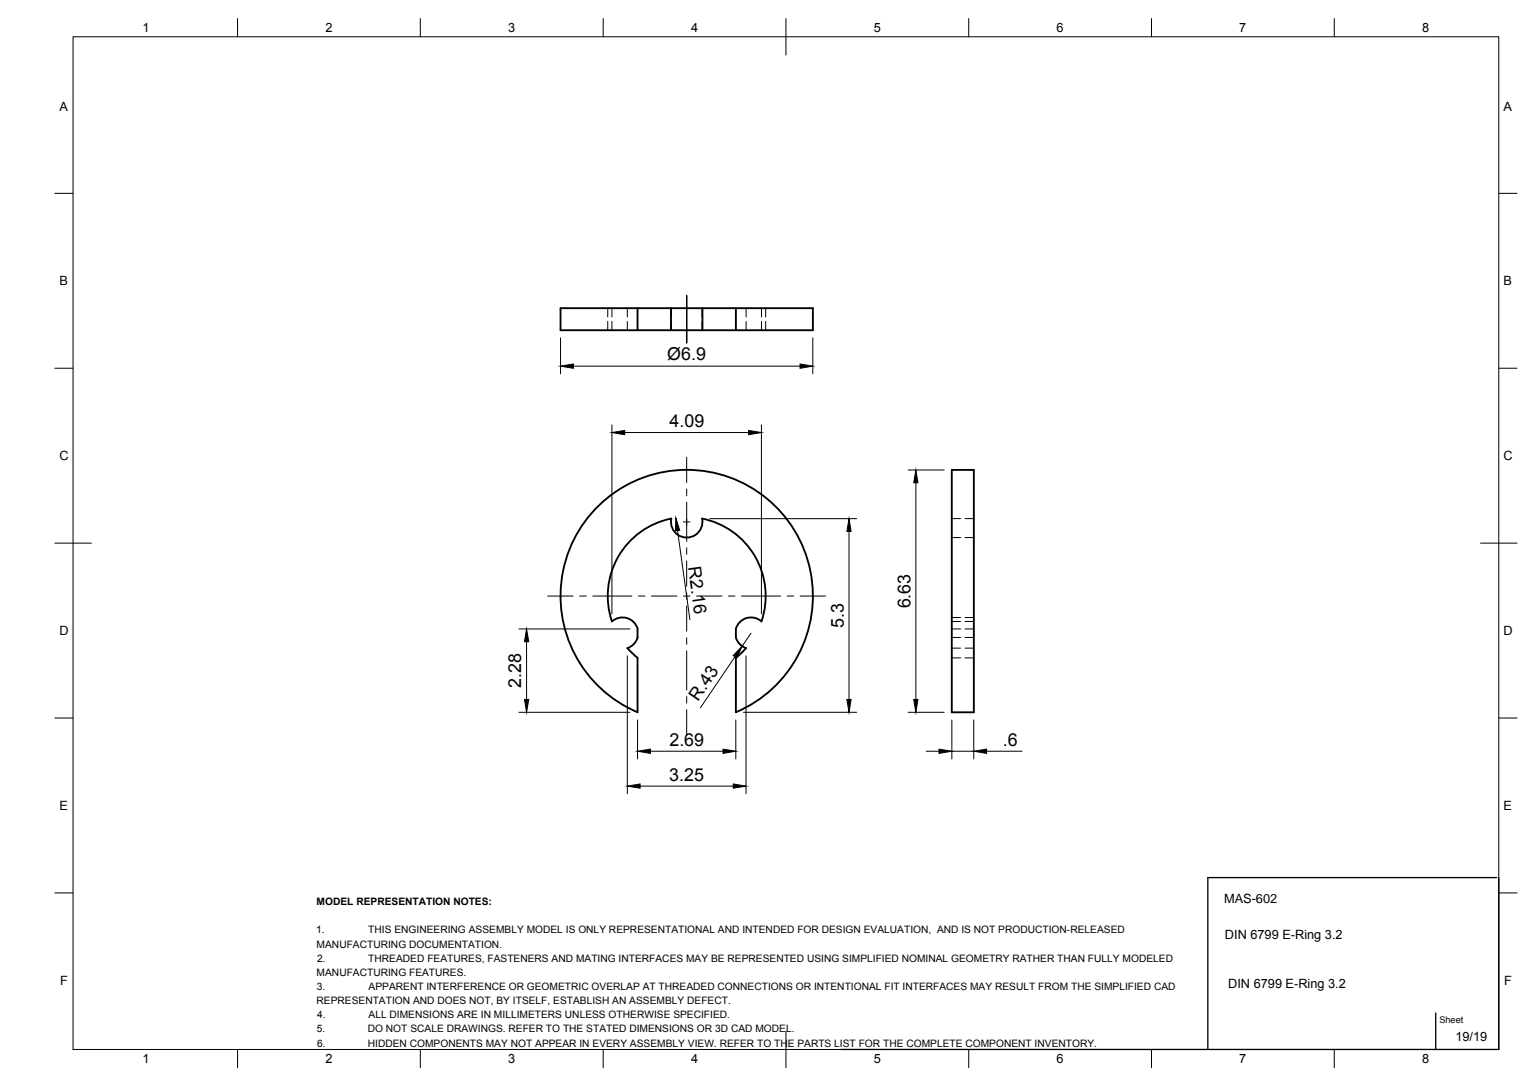
ISO-10303-21;
HEADER;
/* Generated by software containing ST-Developer
 * from STEP Tools, Inc. (www.steptools.com) 
 */

FILE_DESCRIPTION(
/* description */ (''),
/* implementation_level */ '2;1');

FILE_NAME(
/* name */ 'DIN 6799 E-Ring 3.2.step',
/* time_stamp */ '2026-10-15T14:42:47-07:00',
/* author */ (''),
/* organization */ (''),
/* preprocessor_version */ 'ST-DEVELOPER v20.2',
/* originating_system */ 'Autodesk Translation Framework v15.15.0.0',
/* authorisation */ '');

FILE_SCHEMA (('AUTOMOTIVE_DESIGN { 1 0 10303 214 3 1 1 }'));
ENDSEC;

DATA;
#10=MECHANICAL_DESIGN_GEOMETRIC_PRESENTATION_REPRESENTATION('',(#251),#85789);
#215=SHAPE_REPRESENTATION_RELATIONSHIP('SRR','None',#85880,#233);
#233=ADVANCED_BREP_SHAPE_REPRESENTATION('',(#269),#85788);
#251=STYLED_ITEM('',(#85978),#269);
#269=MANIFOLD_SOLID_BREP('Body1',#9898);
#1193=PLANE('',#10893);
#1194=PLANE('',#10894);
#1195=PLANE('',#10895);
#1196=PLANE('',#10896);
#1197=PLANE('',#10912);
#1198=PLANE('',#10928);
#1713=LINE('',#85637,#2249);
#1714=LINE('',#85639,#2250);
#1715=LINE('',#85641,#2251);
#1716=LINE('',#85642,#2252);
#1717=LINE('',#85646,#2253);
#1718=LINE('',#85648,#2254);
#1719=LINE('',#85650,#2255);
#1720=LINE('',#85651,#2256);
#1721=LINE('',#85655,#2257);
#1722=LINE('',#85657,#2258);
#1723=LINE('',#85659,#2259);
#1724=LINE('',#85660,#2260);
#1725=LINE('',#85664,#2261);
#1726=LINE('',#85666,#2262);
#1727=LINE('',#85668,#2263);
#1728=LINE('',#85669,#2264);
#1729=LINE('',#85674,#2265);
#1730=LINE('',#85680,#2266);
#1731=LINE('',#85686,#2267);
#1732=LINE('',#85692,#2268);
#1733=LINE('',#85710,#2269);
#1734=LINE('',#85714,#2270);
#2249=VECTOR('',#13065,1.);
#2250=VECTOR('',#13066,1.);
#2251=VECTOR('',#13067,1.);
#2252=VECTOR('',#13068,1.);
#2253=VECTOR('',#13071,1.);
#2254=VECTOR('',#13072,1.);
#2255=VECTOR('',#13073,1.);
#2256=VECTOR('',#13074,1.);
#2257=VECTOR('',#13077,1.);
#2258=VECTOR('',#13078,1.);
#2259=VECTOR('',#13079,1.);
#2260=VECTOR('',#13080,1.);
#2261=VECTOR('',#13083,1.);
#2262=VECTOR('',#13084,1.);
#2263=VECTOR('',#13085,1.);
#2264=VECTOR('',#13086,1.);
#2265=VECTOR('',#13091,1.);
#2266=VECTOR('',#13098,1.);
#2267=VECTOR('',#13105,1.);
#2268=VECTOR('',#13112,1.);
#2269=VECTOR('',#13141,1.);
#2270=VECTOR('',#13146,1.);
#2392=CYLINDRICAL_SURFACE('',#10897,0.04298125);
#2393=CYLINDRICAL_SURFACE('',#10900,0.04298125);
#2394=CYLINDRICAL_SURFACE('',#10903,0.04298125);
#2395=CYLINDRICAL_SURFACE('',#10906,0.04298125);
#2396=CYLINDRICAL_SURFACE('',#10909,0.2159625);
#2397=CYLINDRICAL_SURFACE('',#10918,0.2159625);
#2398=CYLINDRICAL_SURFACE('',#10920,0.2159625);
#2399=CYLINDRICAL_SURFACE('',#10922,0.04298125);
#2400=CYLINDRICAL_SURFACE('',#10924,0.2159625);
#2401=CYLINDRICAL_SURFACE('',#10926,0.345);
#2887=FACE_OUTER_BOUND('',#3477,.T.);
#2888=FACE_OUTER_BOUND('',#3478,.T.);
#2889=FACE_OUTER_BOUND('',#3479,.T.);
#2890=FACE_OUTER_BOUND('',#3480,.T.);
#2891=FACE_OUTER_BOUND('',#3481,.T.);
#2892=FACE_OUTER_BOUND('',#3482,.T.);
#2893=FACE_OUTER_BOUND('',#3483,.T.);
#2894=FACE_OUTER_BOUND('',#3484,.T.);
#2895=FACE_OUTER_BOUND('',#3485,.T.);
#2896=FACE_OUTER_BOUND('',#3486,.T.);
#2897=FACE_OUTER_BOUND('',#3487,.T.);
#2898=FACE_OUTER_BOUND('',#3488,.T.);
#2899=FACE_OUTER_BOUND('',#3489,.T.);
#2900=FACE_OUTER_BOUND('',#3490,.T.);
#2901=FACE_OUTER_BOUND('',#3491,.T.);
#2902=FACE_OUTER_BOUND('',#3492,.T.);
#3477=EDGE_LOOP('',(#9291,#9292,#9293,#9294));
#3478=EDGE_LOOP('',(#9295,#9296,#9297,#9298));
#3479=EDGE_LOOP('',(#9299,#9300,#9301,#9302));
#3480=EDGE_LOOP('',(#9303,#9304,#9305,#9306));
#3481=EDGE_LOOP('',(#9307,#9308,#9309,#9310));
#3482=EDGE_LOOP('',(#9311,#9312,#9313,#9314));
#3483=EDGE_LOOP('',(#9315,#9316,#9317,#9318));
#3484=EDGE_LOOP('',(#9319,#9320,#9321,#9322));
#3485=EDGE_LOOP('',(#9323,#9324,#9325,#9326));
#3486=EDGE_LOOP('',(#9327,#9328,#9329,#9330,#9331,#9332,#9333,#9334,#9335,
#9336,#9337,#9338,#9339,#9340));
#3487=EDGE_LOOP('',(#9341,#9342,#9343,#9344));
#3488=EDGE_LOOP('',(#9345,#9346,#9347,#9348));
#3489=EDGE_LOOP('',(#9349,#9350,#9351,#9352));
#3490=EDGE_LOOP('',(#9353,#9354,#9355,#9356));
#3491=EDGE_LOOP('',(#9357,#9358,#9359,#9360));
#3492=EDGE_LOOP('',(#9361,#9362,#9363,#9364,#9365,#9366,#9367,#9368,#9369,
#9370,#9371,#9372,#9373,#9374));
#3875=CIRCLE('',#10898,0.04298125);
#3876=CIRCLE('',#10899,0.04298125);
#3877=CIRCLE('',#10901,0.04298125);
#3878=CIRCLE('',#10902,0.04298125);
#3879=CIRCLE('',#10904,0.04298125);
#3880=CIRCLE('',#10905,0.04298125);
#3881=CIRCLE('',#10907,0.04298125);
#3882=CIRCLE('',#10908,0.04298125);
#3883=CIRCLE('',#10910,0.2159625);
#3884=CIRCLE('',#10911,0.2159625);
#3885=CIRCLE('',#10913,0.2159625);
#3886=CIRCLE('',#10914,0.04298125);
#3887=CIRCLE('',#10915,0.2159625);
#3888=CIRCLE('',#10916,0.345);
#3889=CIRCLE('',#10917,0.2159625);
#3890=CIRCLE('',#10919,0.2159625);
#3891=CIRCLE('',#10921,0.2159625);
#3892=CIRCLE('',#10923,0.04298125);
#3893=CIRCLE('',#10925,0.2159625);
#3894=CIRCLE('',#10927,0.345);
#4907=VERTEX_POINT('',#85635);
#4908=VERTEX_POINT('',#85636);
#4909=VERTEX_POINT('',#85638);
#4910=VERTEX_POINT('',#85640);
#4911=VERTEX_POINT('',#85644);
#4912=VERTEX_POINT('',#85645);
#4913=VERTEX_POINT('',#85647);
#4914=VERTEX_POINT('',#85649);
#4915=VERTEX_POINT('',#85653);
#4916=VERTEX_POINT('',#85654);
#4917=VERTEX_POINT('',#85656);
#4918=VERTEX_POINT('',#85658);
#4919=VERTEX_POINT('',#85662);
#4920=VERTEX_POINT('',#85663);
#4921=VERTEX_POINT('',#85665);
#4922=VERTEX_POINT('',#85667);
#4923=VERTEX_POINT('',#85671);
#4924=VERTEX_POINT('',#85673);
#4925=VERTEX_POINT('',#85677);
#4926=VERTEX_POINT('',#85679);
#4927=VERTEX_POINT('',#85683);
#4928=VERTEX_POINT('',#85685);
#4929=VERTEX_POINT('',#85689);
#4930=VERTEX_POINT('',#85691);
#4931=VERTEX_POINT('',#85698);
#4932=VERTEX_POINT('',#85700);
#4933=VERTEX_POINT('',#85708);
#4934=VERTEX_POINT('',#85712);
#6373=EDGE_CURVE('',#4907,#4908,#1713,.T.);
#6374=EDGE_CURVE('',#4909,#4907,#1714,.T.);
#6375=EDGE_CURVE('',#4910,#4909,#1715,.T.);
#6376=EDGE_CURVE('',#4908,#4910,#1716,.T.);
#6377=EDGE_CURVE('',#4911,#4912,#1717,.T.);
#6378=EDGE_CURVE('',#4913,#4911,#1718,.T.);
#6379=EDGE_CURVE('',#4914,#4913,#1719,.T.);
#6380=EDGE_CURVE('',#4912,#4914,#1720,.T.);
#6381=EDGE_CURVE('',#4915,#4916,#1721,.T.);
#6382=EDGE_CURVE('',#4917,#4915,#1722,.T.);
#6383=EDGE_CURVE('',#4918,#4917,#1723,.T.);
#6384=EDGE_CURVE('',#4916,#4918,#1724,.T.);
#6385=EDGE_CURVE('',#4919,#4920,#1725,.T.);
#6386=EDGE_CURVE('',#4921,#4919,#1726,.T.);
#6387=EDGE_CURVE('',#4922,#4921,#1727,.T.);
#6388=EDGE_CURVE('',#4920,#4922,#1728,.T.);
#6389=EDGE_CURVE('',#4923,#4913,#3875,.T.);
#6390=EDGE_CURVE('',#4924,#4923,#1729,.T.);
#6391=EDGE_CURVE('',#4924,#4914,#3876,.T.);
#6392=EDGE_CURVE('',#4912,#4925,#3877,.T.);
#6393=EDGE_CURVE('',#4925,#4926,#1730,.T.);
#6394=EDGE_CURVE('',#4911,#4926,#3878,.T.);
#6395=EDGE_CURVE('',#4927,#4921,#3879,.T.);
#6396=EDGE_CURVE('',#4928,#4927,#1731,.T.);
#6397=EDGE_CURVE('',#4928,#4922,#3880,.T.);
#6398=EDGE_CURVE('',#4920,#4929,#3881,.T.);
#6399=EDGE_CURVE('',#4929,#4930,#1732,.T.);
#6400=EDGE_CURVE('',#4919,#4930,#3882,.T.);
#6401=EDGE_CURVE('',#4916,#4928,#3883,.T.);
#6402=EDGE_CURVE('',#4915,#4927,#3884,.T.);
#6403=EDGE_CURVE('',#4931,#4924,#3885,.T.);
#6404=EDGE_CURVE('',#4932,#4931,#3886,.T.);
#6405=EDGE_CURVE('',#4929,#4932,#3887,.T.);
#6406=EDGE_CURVE('',#4909,#4918,#3888,.T.);
#6407=EDGE_CURVE('',#4925,#4907,#3889,.T.);
#6408=EDGE_CURVE('',#4926,#4908,#3890,.T.);
#6409=EDGE_CURVE('',#4933,#4923,#3891,.T.);
#6410=EDGE_CURVE('',#4931,#4933,#1733,.T.);
#6411=EDGE_CURVE('',#4934,#4933,#3892,.T.);
#6412=EDGE_CURVE('',#4932,#4934,#1734,.T.);
#6413=EDGE_CURVE('',#4930,#4934,#3893,.T.);
#6414=EDGE_CURVE('',#4910,#4917,#3894,.T.);
#9291=ORIENTED_EDGE('',*,*,#6373,.F.);
#9292=ORIENTED_EDGE('',*,*,#6374,.F.);
#9293=ORIENTED_EDGE('',*,*,#6375,.F.);
#9294=ORIENTED_EDGE('',*,*,#6376,.F.);
#9295=ORIENTED_EDGE('',*,*,#6377,.F.);
#9296=ORIENTED_EDGE('',*,*,#6378,.F.);
#9297=ORIENTED_EDGE('',*,*,#6379,.F.);
#9298=ORIENTED_EDGE('',*,*,#6380,.F.);
#9299=ORIENTED_EDGE('',*,*,#6381,.F.);
#9300=ORIENTED_EDGE('',*,*,#6382,.F.);
#9301=ORIENTED_EDGE('',*,*,#6383,.F.);
#9302=ORIENTED_EDGE('',*,*,#6384,.F.);
#9303=ORIENTED_EDGE('',*,*,#6385,.F.);
#9304=ORIENTED_EDGE('',*,*,#6386,.F.);
#9305=ORIENTED_EDGE('',*,*,#6387,.F.);
#9306=ORIENTED_EDGE('',*,*,#6388,.F.);
#9307=ORIENTED_EDGE('',*,*,#6379,.T.);
#9308=ORIENTED_EDGE('',*,*,#6389,.F.);
#9309=ORIENTED_EDGE('',*,*,#6390,.F.);
#9310=ORIENTED_EDGE('',*,*,#6391,.T.);
#9311=ORIENTED_EDGE('',*,*,#6377,.T.);
#9312=ORIENTED_EDGE('',*,*,#6392,.T.);
#9313=ORIENTED_EDGE('',*,*,#6393,.T.);
#9314=ORIENTED_EDGE('',*,*,#6394,.F.);
#9315=ORIENTED_EDGE('',*,*,#6387,.T.);
#9316=ORIENTED_EDGE('',*,*,#6395,.F.);
#9317=ORIENTED_EDGE('',*,*,#6396,.F.);
#9318=ORIENTED_EDGE('',*,*,#6397,.T.);
#9319=ORIENTED_EDGE('',*,*,#6385,.T.);
#9320=ORIENTED_EDGE('',*,*,#6398,.T.);
#9321=ORIENTED_EDGE('',*,*,#6399,.T.);
#9322=ORIENTED_EDGE('',*,*,#6400,.F.);
#9323=ORIENTED_EDGE('',*,*,#6381,.T.);
#9324=ORIENTED_EDGE('',*,*,#6401,.T.);
#9325=ORIENTED_EDGE('',*,*,#6396,.T.);
#9326=ORIENTED_EDGE('',*,*,#6402,.F.);
#9327=ORIENTED_EDGE('',*,*,#6380,.T.);
#9328=ORIENTED_EDGE('',*,*,#6391,.F.);
#9329=ORIENTED_EDGE('',*,*,#6403,.F.);
#9330=ORIENTED_EDGE('',*,*,#6404,.F.);
#9331=ORIENTED_EDGE('',*,*,#6405,.F.);
#9332=ORIENTED_EDGE('',*,*,#6398,.F.);
#9333=ORIENTED_EDGE('',*,*,#6388,.T.);
#9334=ORIENTED_EDGE('',*,*,#6397,.F.);
#9335=ORIENTED_EDGE('',*,*,#6401,.F.);
#9336=ORIENTED_EDGE('',*,*,#6384,.T.);
#9337=ORIENTED_EDGE('',*,*,#6406,.F.);
#9338=ORIENTED_EDGE('',*,*,#6374,.T.);
#9339=ORIENTED_EDGE('',*,*,#6407,.F.);
#9340=ORIENTED_EDGE('',*,*,#6392,.F.);
#9341=ORIENTED_EDGE('',*,*,#6373,.T.);
#9342=ORIENTED_EDGE('',*,*,#6408,.F.);
#9343=ORIENTED_EDGE('',*,*,#6393,.F.);
#9344=ORIENTED_EDGE('',*,*,#6407,.T.);
#9345=ORIENTED_EDGE('',*,*,#6403,.T.);
#9346=ORIENTED_EDGE('',*,*,#6390,.T.);
#9347=ORIENTED_EDGE('',*,*,#6409,.F.);
#9348=ORIENTED_EDGE('',*,*,#6410,.F.);
#9349=ORIENTED_EDGE('',*,*,#6404,.T.);
#9350=ORIENTED_EDGE('',*,*,#6410,.T.);
#9351=ORIENTED_EDGE('',*,*,#6411,.F.);
#9352=ORIENTED_EDGE('',*,*,#6412,.F.);
#9353=ORIENTED_EDGE('',*,*,#6405,.T.);
#9354=ORIENTED_EDGE('',*,*,#6412,.T.);
#9355=ORIENTED_EDGE('',*,*,#6413,.F.);
#9356=ORIENTED_EDGE('',*,*,#6399,.F.);
#9357=ORIENTED_EDGE('',*,*,#6375,.T.);
#9358=ORIENTED_EDGE('',*,*,#6406,.T.);
#9359=ORIENTED_EDGE('',*,*,#6383,.T.);
#9360=ORIENTED_EDGE('',*,*,#6414,.F.);
#9361=ORIENTED_EDGE('',*,*,#6378,.T.);
#9362=ORIENTED_EDGE('',*,*,#6394,.T.);
#9363=ORIENTED_EDGE('',*,*,#6408,.T.);
#9364=ORIENTED_EDGE('',*,*,#6376,.T.);
#9365=ORIENTED_EDGE('',*,*,#6414,.T.);
#9366=ORIENTED_EDGE('',*,*,#6382,.T.);
#9367=ORIENTED_EDGE('',*,*,#6402,.T.);
#9368=ORIENTED_EDGE('',*,*,#6395,.T.);
#9369=ORIENTED_EDGE('',*,*,#6386,.T.);
#9370=ORIENTED_EDGE('',*,*,#6400,.T.);
#9371=ORIENTED_EDGE('',*,*,#6413,.T.);
#9372=ORIENTED_EDGE('',*,*,#6411,.T.);
#9373=ORIENTED_EDGE('',*,*,#6409,.T.);
#9374=ORIENTED_EDGE('',*,*,#6389,.T.);
#9865=ADVANCED_FACE('',(#2887),#1193,.F.);
#9866=ADVANCED_FACE('',(#2888),#1194,.F.);
#9867=ADVANCED_FACE('',(#2889),#1195,.F.);
#9868=ADVANCED_FACE('',(#2890),#1196,.F.);
#9869=ADVANCED_FACE('',(#2891),#2392,.T.);
#9870=ADVANCED_FACE('',(#2892),#2393,.T.);
#9871=ADVANCED_FACE('',(#2893),#2394,.T.);
#9872=ADVANCED_FACE('',(#2894),#2395,.T.);
#9873=ADVANCED_FACE('',(#2895),#2396,.F.);
#9874=ADVANCED_FACE('',(#2896),#1197,.F.);
#9875=ADVANCED_FACE('',(#2897),#2397,.F.);
#9876=ADVANCED_FACE('',(#2898),#2398,.F.);
#9877=ADVANCED_FACE('',(#2899),#2399,.T.);
#9878=ADVANCED_FACE('',(#2900),#2400,.F.);
#9879=ADVANCED_FACE('',(#2901),#2401,.T.);
#9880=ADVANCED_FACE('',(#2902),#1198,.T.);
#9898=CLOSED_SHELL('',(#9865,#9866,#9867,#9868,#9869,#9870,#9871,#9872,
#9873,#9874,#9875,#9876,#9877,#9878,#9879,#9880));
#10892=AXIS2_PLACEMENT_3D('',#85633,#13061,#13062);
#10893=AXIS2_PLACEMENT_3D('',#85634,#13063,#13064);
#10894=AXIS2_PLACEMENT_3D('',#85643,#13069,#13070);
#10895=AXIS2_PLACEMENT_3D('',#85652,#13075,#13076);
#10896=AXIS2_PLACEMENT_3D('',#85661,#13081,#13082);
#10897=AXIS2_PLACEMENT_3D('',#85670,#13087,#13088);
#10898=AXIS2_PLACEMENT_3D('',#85672,#13089,#13090);
#10899=AXIS2_PLACEMENT_3D('',#85675,#13092,#13093);
#10900=AXIS2_PLACEMENT_3D('',#85676,#13094,#13095);
#10901=AXIS2_PLACEMENT_3D('',#85678,#13096,#13097);
#10902=AXIS2_PLACEMENT_3D('',#85681,#13099,#13100);
#10903=AXIS2_PLACEMENT_3D('',#85682,#13101,#13102);
#10904=AXIS2_PLACEMENT_3D('',#85684,#13103,#13104);
#10905=AXIS2_PLACEMENT_3D('',#85687,#13106,#13107);
#10906=AXIS2_PLACEMENT_3D('',#85688,#13108,#13109);
#10907=AXIS2_PLACEMENT_3D('',#85690,#13110,#13111);
#10908=AXIS2_PLACEMENT_3D('',#85693,#13113,#13114);
#10909=AXIS2_PLACEMENT_3D('',#85694,#13115,#13116);
#10910=AXIS2_PLACEMENT_3D('',#85695,#13117,#13118);
#10911=AXIS2_PLACEMENT_3D('',#85696,#13119,#13120);
#10912=AXIS2_PLACEMENT_3D('',#85697,#13121,#13122);
#10913=AXIS2_PLACEMENT_3D('',#85699,#13123,#13124);
#10914=AXIS2_PLACEMENT_3D('',#85701,#13125,#13126);
#10915=AXIS2_PLACEMENT_3D('',#85702,#13127,#13128);
#10916=AXIS2_PLACEMENT_3D('',#85703,#13129,#13130);
#10917=AXIS2_PLACEMENT_3D('',#85704,#13131,#13132);
#10918=AXIS2_PLACEMENT_3D('',#85705,#13133,#13134);
#10919=AXIS2_PLACEMENT_3D('',#85706,#13135,#13136);
#10920=AXIS2_PLACEMENT_3D('',#85707,#13137,#13138);
#10921=AXIS2_PLACEMENT_3D('',#85709,#13139,#13140);
#10922=AXIS2_PLACEMENT_3D('',#85711,#13142,#13143);
#10923=AXIS2_PLACEMENT_3D('',#85713,#13144,#13145);
#10924=AXIS2_PLACEMENT_3D('',#85715,#13147,#13148);
#10925=AXIS2_PLACEMENT_3D('',#85716,#13149,#13150);
#10926=AXIS2_PLACEMENT_3D('',#85717,#13151,#13152);
#10927=AXIS2_PLACEMENT_3D('',#85718,#13153,#13154);
#10928=AXIS2_PLACEMENT_3D('',#85719,#13155,#13156);
#13061=DIRECTION('axis',(0.,0.,1.));
#13062=DIRECTION('refdir',(1.,0.,0.));
#13063=DIRECTION('center_axis',(0.,1.,0.));
#13064=DIRECTION('ref_axis',(0.,0.,1.));
#13065=DIRECTION('',(1.,0.,0.));
#13066=DIRECTION('',(0.,0.,1.));
#13067=DIRECTION('',(-1.,0.,0.));
#13068=DIRECTION('',(0.,0.,-1.));
#13069=DIRECTION('center_axis',(0.,1.,0.));
#13070=DIRECTION('ref_axis',(0.,0.,1.));
#13071=DIRECTION('',(-1.,0.,0.));
#13072=DIRECTION('',(0.,0.,-1.));
#13073=DIRECTION('',(1.,0.,0.));
#13074=DIRECTION('',(0.,0.,1.));
#13075=DIRECTION('center_axis',(0.,-1.,0.));
#13076=DIRECTION('ref_axis',(0.,0.,-1.));
#13077=DIRECTION('',(-1.,0.,0.));
#13078=DIRECTION('',(0.,0.,1.));
#13079=DIRECTION('',(1.,0.,0.));
#13080=DIRECTION('',(0.,0.,-1.));
#13081=DIRECTION('center_axis',(0.,-1.,0.));
#13082=DIRECTION('ref_axis',(0.,0.,-1.));
#13083=DIRECTION('',(-1.,0.,0.));
#13084=DIRECTION('',(0.,0.,1.));
#13085=DIRECTION('',(1.,0.,0.));
#13086=DIRECTION('',(0.,0.,-1.));
#13087=DIRECTION('center_axis',(1.,0.,0.));
#13088=DIRECTION('ref_axis',(0.,-0.279568819041295,0.960125656057506));
#13089=DIRECTION('center_axis',(1.,0.,0.));
#13090=DIRECTION('ref_axis',(0.,0.,-1.));
#13091=DIRECTION('',(1.,0.,0.));
#13092=DIRECTION('center_axis',(1.,0.,0.));
#13093=DIRECTION('ref_axis',(0.,0.,-1.));
#13094=DIRECTION('center_axis',(1.,0.,0.));
#13095=DIRECTION('ref_axis',(0.,0.,-1.));
#13096=DIRECTION('center_axis',(1.,0.,0.));
#13097=DIRECTION('ref_axis',(0.,0.,-1.));
#13098=DIRECTION('',(1.,0.,0.));
#13099=DIRECTION('center_axis',(1.,0.,0.));
#13100=DIRECTION('ref_axis',(0.,0.,-1.));
#13101=DIRECTION('center_axis',(1.,0.,0.));
#13102=DIRECTION('ref_axis',(0.,0.,-1.));
#13103=DIRECTION('center_axis',(1.,0.,0.));
#13104=DIRECTION('ref_axis',(0.,0.,-1.));
#13105=DIRECTION('',(1.,0.,0.));
#13106=DIRECTION('center_axis',(1.,0.,0.));
#13107=DIRECTION('ref_axis',(0.,0.,-1.));
#13108=DIRECTION('center_axis',(1.,0.,0.));
#13109=DIRECTION('ref_axis',(0.,0.279568819041297,0.960125656057505));
#13110=DIRECTION('center_axis',(1.,0.,0.));
#13111=DIRECTION('ref_axis',(0.,0.,-1.));
#13112=DIRECTION('',(1.,0.,0.));
#13113=DIRECTION('center_axis',(1.,0.,0.));
#13114=DIRECTION('ref_axis',(0.,0.,-1.));
#13115=DIRECTION('center_axis',(1.,0.,0.));
#13116=DIRECTION('ref_axis',(0.,0.,-1.));
#13117=DIRECTION('center_axis',(-1.,0.,0.));
#13118=DIRECTION('ref_axis',(0.,0.,-1.));
#13119=DIRECTION('center_axis',(-1.,0.,0.));
#13120=DIRECTION('ref_axis',(0.,0.,-1.));
#13121=DIRECTION('center_axis',(1.,0.,0.));
#13122=DIRECTION('ref_axis',(0.,0.,-1.));
#13123=DIRECTION('center_axis',(-1.,0.,0.));
#13124=DIRECTION('ref_axis',(0.,0.,-1.));
#13125=DIRECTION('center_axis',(1.,0.,0.));
#13126=DIRECTION('ref_axis',(0.,0.,-1.));
#13127=DIRECTION('center_axis',(-1.,0.,0.));
#13128=DIRECTION('ref_axis',(0.,0.,-1.));
#13129=DIRECTION('center_axis',(1.,0.,0.));
#13130=DIRECTION('ref_axis',(0.,0.,-1.));
#13131=DIRECTION('center_axis',(-1.,0.,0.));
#13132=DIRECTION('ref_axis',(0.,0.,-1.));
#13133=DIRECTION('center_axis',(1.,0.,0.));
#13134=DIRECTION('ref_axis',(0.,0.,-1.));
#13135=DIRECTION('center_axis',(-1.,0.,0.));
#13136=DIRECTION('ref_axis',(0.,0.,-1.));
#13137=DIRECTION('center_axis',(1.,0.,0.));
#13138=DIRECTION('ref_axis',(0.,0.,-1.));
#13139=DIRECTION('center_axis',(-1.,0.,0.));
#13140=DIRECTION('ref_axis',(0.,0.,-1.));
#13141=DIRECTION('',(1.,0.,0.));
#13142=DIRECTION('center_axis',(1.,0.,0.));
#13143=DIRECTION('ref_axis',(0.,0.,-1.));
#13144=DIRECTION('center_axis',(1.,0.,0.));
#13145=DIRECTION('ref_axis',(0.,0.,-1.));
#13146=DIRECTION('',(1.,0.,0.));
#13147=DIRECTION('center_axis',(1.,0.,0.));
#13148=DIRECTION('ref_axis',(0.,0.,-1.));
#13149=DIRECTION('center_axis',(-1.,0.,0.));
#13150=DIRECTION('ref_axis',(0.,0.,-1.));
#13151=DIRECTION('center_axis',(1.,0.,0.));
#13152=DIRECTION('ref_axis',(0.,1.22464679914735E-16,1.));
#13153=DIRECTION('center_axis',(1.,0.,0.));
#13154=DIRECTION('ref_axis',(0.,0.,-1.));
#13155=DIRECTION('center_axis',(1.,0.,0.));
#13156=DIRECTION('ref_axis',(0.,0.,-1.));
#85633=CARTESIAN_POINT('',(0.,0.,0.));
#85634=CARTESIAN_POINT('Origin',(0.,0.1344,-0.69));
#85635=CARTESIAN_POINT('',(0.,0.1344,-0.169045678460734));
#85636=CARTESIAN_POINT('',(0.06,0.1344,-0.169045678460734));
#85637=CARTESIAN_POINT('',(0.,0.1344,-0.169045678460734));
#85638=CARTESIAN_POINT('',(0.,0.1344,-0.31774461443115));
#85639=CARTESIAN_POINT('',(0.,0.1344,-0.345));
#85640=CARTESIAN_POINT('',(0.06,0.1344,-0.31774461443115));
#85641=CARTESIAN_POINT('',(0.,0.1344,-0.31774461443115));
#85642=CARTESIAN_POINT('',(0.06,0.1344,-0.345));
#85643=CARTESIAN_POINT('Origin',(0.,0.1344,-0.69));
#85644=CARTESIAN_POINT('',(0.06,0.1344,-0.11308850359562));
#85645=CARTESIAN_POINT('',(0.,0.1344,-0.11308850359562));
#85646=CARTESIAN_POINT('',(0.,0.1344,-0.11308850359562));
#85647=CARTESIAN_POINT('',(0.06,0.1344,-0.0898927464043797));
#85648=CARTESIAN_POINT('',(0.06,0.1344,-0.345));
#85649=CARTESIAN_POINT('',(0.,0.1344,-0.0898927464043797));
#85650=CARTESIAN_POINT('',(0.,0.1344,-0.0898927464043797));
#85651=CARTESIAN_POINT('',(0.,0.1344,-0.345));
#85652=CARTESIAN_POINT('Origin',(0.,-0.1344,-0.048));
#85653=CARTESIAN_POINT('',(0.06,-0.1344,-0.169045678460734));
#85654=CARTESIAN_POINT('',(0.,-0.1344,-0.169045678460734));
#85655=CARTESIAN_POINT('',(0.,-0.1344,-0.169045678460734));
#85656=CARTESIAN_POINT('',(0.06,-0.1344,-0.31774461443115));
#85657=CARTESIAN_POINT('',(0.06,-0.1344,-0.024));
#85658=CARTESIAN_POINT('',(0.,-0.1344,-0.31774461443115));
#85659=CARTESIAN_POINT('',(0.,-0.1344,-0.31774461443115));
#85660=CARTESIAN_POINT('',(0.,-0.1344,-0.024));
#85661=CARTESIAN_POINT('Origin',(0.,-0.1344,-0.048));
#85662=CARTESIAN_POINT('',(0.06,-0.1344,-0.0898927464043798));
#85663=CARTESIAN_POINT('',(0.,-0.1344,-0.0898927464043798));
#85664=CARTESIAN_POINT('',(0.,-0.1344,-0.0898927464043798));
#85665=CARTESIAN_POINT('',(0.06,-0.1344,-0.11308850359562));
#85666=CARTESIAN_POINT('',(0.06,-0.1344,-0.024));
#85667=CARTESIAN_POINT('',(0.,-0.1344,-0.11308850359562));
#85668=CARTESIAN_POINT('',(0.,-0.1344,-0.11308850359562));
#85669=CARTESIAN_POINT('',(0.,-0.1344,-0.024));
#85670=CARTESIAN_POINT('Origin',(0.,0.17578691899192,-0.101490625));
#85671=CARTESIAN_POINT('',(0.06,0.204478107495771,-0.0694874446299335));
#85672=CARTESIAN_POINT('Origin',(0.06,0.17578691899192,-0.101490625));
#85673=CARTESIAN_POINT('',(0.,0.204478107495771,-0.0694874446299335));
#85674=CARTESIAN_POINT('',(0.,0.204478107495771,-0.0694874446299335));
#85675=CARTESIAN_POINT('Origin',(0.,0.17578691899192,-0.101490625));
#85676=CARTESIAN_POINT('Origin',(0.,0.17578691899192,-0.101490625));
#85677=CARTESIAN_POINT('',(0.,0.162416946041472,-0.142339513294136));
#85678=CARTESIAN_POINT('Origin',(0.,0.17578691899192,-0.101490625));
#85679=CARTESIAN_POINT('',(0.06,0.162416946041472,-0.142339513294136));
#85680=CARTESIAN_POINT('',(0.,0.162416946041472,-0.142339513294136));
#85681=CARTESIAN_POINT('Origin',(0.06,0.17578691899192,-0.101490625));
#85682=CARTESIAN_POINT('Origin',(0.,-0.17578691899192,-0.101490625));
#85683=CARTESIAN_POINT('',(0.06,-0.162416946041472,-0.142339513294136));
#85684=CARTESIAN_POINT('Origin',(0.06,-0.17578691899192,-0.101490625));
#85685=CARTESIAN_POINT('',(0.,-0.162416946041472,-0.142339513294136));
#85686=CARTESIAN_POINT('',(0.,-0.162416946041472,-0.142339513294136));
#85687=CARTESIAN_POINT('Origin',(0.,-0.17578691899192,-0.101490625));
#85688=CARTESIAN_POINT('Origin',(0.,-0.17578691899192,-0.101490625));
#85689=CARTESIAN_POINT('',(0.,-0.204478107495771,-0.0694874446299334));
#85690=CARTESIAN_POINT('Origin',(0.,-0.17578691899192,-0.101490625));
#85691=CARTESIAN_POINT('',(0.06,-0.204478107495771,-0.0694874446299334));
#85692=CARTESIAN_POINT('',(0.,-0.204478107495771,-0.0694874446299334));
#85693=CARTESIAN_POINT('Origin',(0.06,-0.17578691899192,-0.101490625));
#85694=CARTESIAN_POINT('Origin',(0.,0.,0.));
#85695=CARTESIAN_POINT('Origin',(0.,0.,0.));
#85696=CARTESIAN_POINT('Origin',(0.06,0.,0.));
#85697=CARTESIAN_POINT('Origin',(0.,0.,0.));
#85698=CARTESIAN_POINT('',(0.,0.0420611614542984,0.211826957924069));
#85699=CARTESIAN_POINT('Origin',(0.,0.,0.));
#85700=CARTESIAN_POINT('',(0.,-0.0420611614542984,0.211826957924069));
#85701=CARTESIAN_POINT('Origin',(0.,1.24290169049714E-17,0.20298125));
#85702=CARTESIAN_POINT('Origin',(0.,0.,0.));
#85703=CARTESIAN_POINT('Origin',(0.,0.,0.));
#85704=CARTESIAN_POINT('Origin',(0.,0.,0.));
#85705=CARTESIAN_POINT('Origin',(0.,0.,0.));
#85706=CARTESIAN_POINT('Origin',(0.06,0.,0.));
#85707=CARTESIAN_POINT('Origin',(0.,0.,0.));
#85708=CARTESIAN_POINT('',(0.06,0.0420611614542984,0.211826957924069));
#85709=CARTESIAN_POINT('Origin',(0.06,0.,0.));
#85710=CARTESIAN_POINT('',(0.,0.0420611614542984,0.211826957924069));
#85711=CARTESIAN_POINT('Origin',(0.,1.24290169049714E-17,0.20298125));
#85712=CARTESIAN_POINT('',(0.06,-0.0420611614542984,0.211826957924069));
#85713=CARTESIAN_POINT('Origin',(0.06,1.24290169049714E-17,0.20298125));
#85714=CARTESIAN_POINT('',(0.,-0.0420611614542984,0.211826957924069));
#85715=CARTESIAN_POINT('Origin',(0.,0.,0.));
#85716=CARTESIAN_POINT('Origin',(0.06,0.,0.));
#85717=CARTESIAN_POINT('Origin',(0.,0.,0.));
#85718=CARTESIAN_POINT('Origin',(0.06,0.,0.));
#85719=CARTESIAN_POINT('Origin',(0.06,0.,0.));
#85768=UNCERTAINTY_MEASURE_WITH_UNIT(LENGTH_MEASURE(0.001),#85790,
'DISTANCE_ACCURACY_VALUE',
'Maximum model space distance between geometric entities at asserted c
onnectivities');
#85769=UNCERTAINTY_MEASURE_WITH_UNIT(LENGTH_MEASURE(0.001),#85790,
'DISTANCE_ACCURACY_VALUE',
'Maximum model space distance between geometric entities at asserted c
onnectivities');
#85788=(
GEOMETRIC_REPRESENTATION_CONTEXT(3)
GLOBAL_UNCERTAINTY_ASSIGNED_CONTEXT((#85768))
GLOBAL_UNIT_ASSIGNED_CONTEXT((#85790,#85792,#85793))
REPRESENTATION_CONTEXT('','3D')
);
#85789=(
GEOMETRIC_REPRESENTATION_CONTEXT(3)
GLOBAL_UNCERTAINTY_ASSIGNED_CONTEXT((#85769))
GLOBAL_UNIT_ASSIGNED_CONTEXT((#85790,#85792,#85793))
REPRESENTATION_CONTEXT('','3D')
);
#85790=(
LENGTH_UNIT()
NAMED_UNIT(*)
SI_UNIT(.CENTI.,.METRE.)
);
#85792=(
NAMED_UNIT(*)
PLANE_ANGLE_UNIT()
SI_UNIT($,.RADIAN.)
);
#85793=(
NAMED_UNIT(*)
SI_UNIT($,.STERADIAN.)
SOLID_ANGLE_UNIT()
);
#85812=SHAPE_DEFINITION_REPRESENTATION(#85831,#85880);
#85831=PRODUCT_DEFINITION_SHAPE('',$,#85900);
#85880=SHAPE_REPRESENTATION('',(#10892),#85788);
#85881=PRODUCT_DEFINITION_CONTEXT('part definition',#85940,'design');
#85900=PRODUCT_DEFINITION('DIN 6799 E-Ring 3.2','DIN 6799 E-Ring 3.2',#85919,
#85881);
#85919=PRODUCT_DEFINITION_FORMATION('',$,#85960);
#85940=APPLICATION_CONTEXT(
'Core Data for Automotive Mechanical Design Process');
#85941=PRODUCT_CONTEXT('part definition',#85940,'mechanical');
#85960=PRODUCT('DIN 6799 E-Ring 3.2','DIN 6799 E-Ring 3.2',$,(#85941));
#85978=PRESENTATION_STYLE_ASSIGNMENT((#85996));
#85996=SURFACE_STYLE_USAGE(.BOTH.,#86014);
#86014=SURFACE_SIDE_STYLE('',(#86032));
#86032=SURFACE_STYLE_FILL_AREA(#86050);
#86050=FILL_AREA_STYLE('Opaque(198,202,207)',(#86068));
#86068=FILL_AREA_STYLE_COLOUR('Opaque(198,202,207)',#86086);
#86086=COLOUR_RGB('Opaque(198,202,207)', 0.08235294, 0.09019608, 0.10196078);
ENDSEC;
END-ISO-10303-21;
